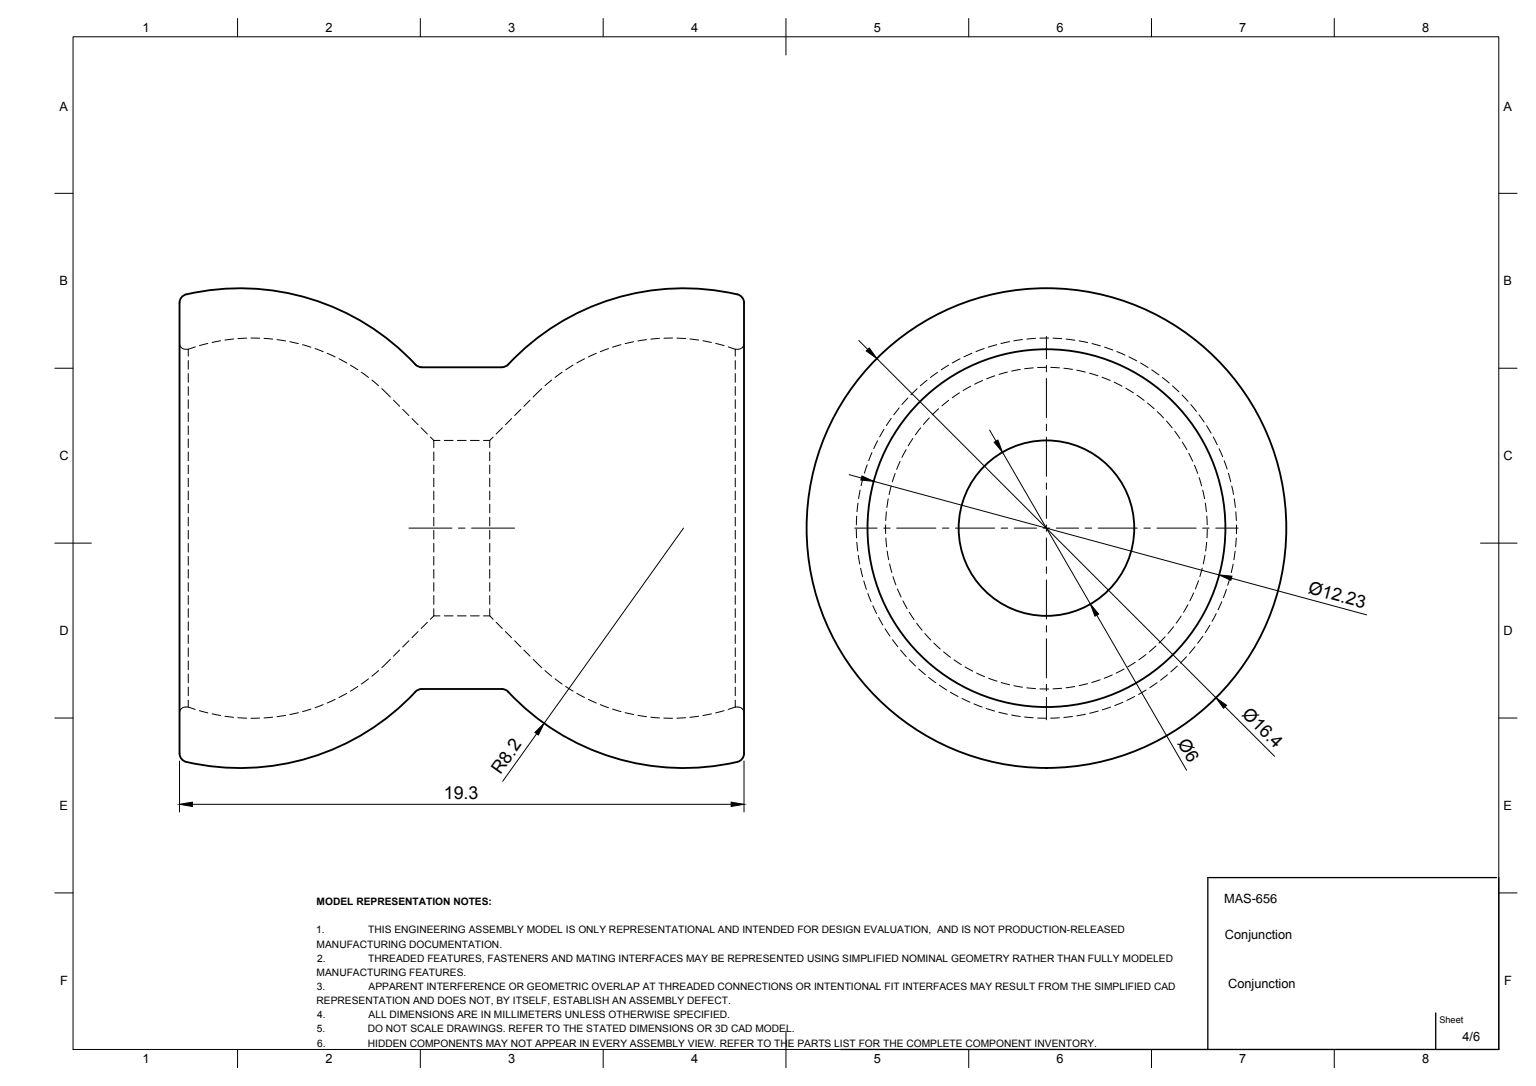
ISO-10303-21;
HEADER;
FILE_DESCRIPTION((''),'2;1');
FILE_NAME('Conjunction.step','2026-10-09T09:41:22-07:00',(''),(''),'','','');
FILE_SCHEMA (('AUTOMOTIVE_DESIGN { 1 0 10303 214 3 1 1 }'));
ENDSEC;
DATA;
#10=MECHANICAL_DESIGN_GEOMETRIC_PRESENTATION_REPRESENTATION('',(#73),#4304);
#65=SHAPE_REPRESENTATION_RELATIONSHIP('SRR','None',#4331,#69) ;
#69=ADVANCED_BREP_SHAPE_REPRESENTATION('',(#79),#4300) ;
#73=STYLED_ITEM('',(#4360),#79) ;
#79=MANIFOLD_SOLID_BREP('Body1',#2162) ;
#85=FACE_BOUND('',#630,.T.) ;
#86=FACE_BOUND('',#634,.T.) ;
#117=PLANE('',#2257) ;
#118=PLANE('',#2264) ;
#161=TOROIDAL_SURFACE('',#2228,7.69960814153059,0.300000000000023) ;
#162=TOROIDAL_SURFACE('',#2233,7.69960814153059,0.300000000000023) ;
#163=TOROIDAL_SURFACE('',#2242,5.80000000000044,0.300000000000023) ;
#164=TOROIDAL_SURFACE('',#2253,5.80000000000044,0.300000000000023) ;
#165=TOROIDAL_SURFACE('',#2259,6.31637147335048,0.200000000000015) ;
#166=TOROIDAL_SURFACE('',#2266,6.31637147335048,0.200000000000015) ;
#177=CYLINDRICAL_SURFACE('',#2221,3.00000000000023) ;
#178=CYLINDRICAL_SURFACE('',#2250,5.50000000000042) ;
#179=CYLINDRICAL_SURFACE('',#2255,6.11637147335047) ;
#180=CYLINDRICAL_SURFACE('',#2261,6.11637147335047) ;
#223=LINE('',#3294,#342) ;
#224=LINE('',#3298,#343) ;
#225=LINE('',#3301,#344) ;
#226=LINE('',#3343,#345) ;
#227=LINE('',#3351,#346) ;
#228=LINE('',#3363,#347) ;
#342=VECTOR('',#2546,3.00000000000023) ;
#343=VECTOR('',#2551,3.00000000000023) ;
#344=VECTOR('',#2554,3.00000000000023) ;
#345=VECTOR('',#2609,5.50000000000042) ;
#346=VECTOR('',#2620,6.11637147335047) ;
#347=VECTOR('',#2637,6.11637147335047) ;
#461=CONICAL_SURFACE('',#2219,3.00000000000023,0.785398163397) ;
#462=CONICAL_SURFACE('',#2223,3.00000000000023,0.785398163397) ;
#480=FACE_OUTER_BOUND('',#616,.T.) ;
#481=FACE_OUTER_BOUND('',#617,.T.) ;
#482=FACE_OUTER_BOUND('',#618,.T.) ;
#483=FACE_OUTER_BOUND('',#619,.T.) ;
#484=FACE_OUTER_BOUND('',#620,.T.) ;
#485=FACE_OUTER_BOUND('',#621,.T.) ;
#486=FACE_OUTER_BOUND('',#622,.T.) ;
#487=FACE_OUTER_BOUND('',#623,.T.) ;
#488=FACE_OUTER_BOUND('',#624,.T.) ;
#489=FACE_OUTER_BOUND('',#625,.T.) ;
#490=FACE_OUTER_BOUND('',#626,.T.) ;
#491=FACE_OUTER_BOUND('',#627,.T.) ;
#492=FACE_OUTER_BOUND('',#628,.T.) ;
#493=FACE_OUTER_BOUND('',#629,.T.) ;
#494=FACE_OUTER_BOUND('',#631,.T.) ;
#495=FACE_OUTER_BOUND('',#632,.T.) ;
#496=FACE_OUTER_BOUND('',#633,.T.) ;
#497=FACE_OUTER_BOUND('',#635,.T.) ;
#616=EDGE_LOOP('',(#1431,#1432,#1433,#1434)) ;
#617=EDGE_LOOP('',(#1435,#1436,#1437,#1438)) ;
#618=EDGE_LOOP('',(#1439,#1440,#1441,#1442)) ;
#619=EDGE_LOOP('',(#1443,#1444,#1445,#1446)) ;
#620=EDGE_LOOP('',(#1447,#1448,#1449,#1450)) ;
#621=EDGE_LOOP('',(#1451,#1452,#1453,#1454,#1455)) ;
#622=EDGE_LOOP('',(#1456,#1457,#1458,#1459,#1460)) ;
#623=EDGE_LOOP('',(#1461,#1462,#1463,#1464,#1465,#1466)) ;
#624=EDGE_LOOP('',(#1467,#1468,#1469,#1470,#1471,#1472)) ;
#625=EDGE_LOOP('',(#1473,#1474,#1475,#1476,#1477,#1478)) ;
#626=EDGE_LOOP('',(#1479,#1480,#1481,#1482,#1483,#1484)) ;
#627=EDGE_LOOP('',(#1485,#1486,#1487,#1488,#1489,#1490)) ;
#628=EDGE_LOOP('',(#1491,#1492,#1493,#1494)) ;
#629=EDGE_LOOP('',(#1495)) ;
#630=EDGE_LOOP('',(#1496)) ;
#631=EDGE_LOOP('',(#1497,#1498,#1499,#1500)) ;
#632=EDGE_LOOP('',(#1501,#1502,#1503,#1504,#1505)) ;
#633=EDGE_LOOP('',(#1506)) ;
#634=EDGE_LOOP('',(#1507)) ;
#635=EDGE_LOOP('',(#1508,#1509,#1510,#1511,#1512)) ;
#784=CIRCLE('',#2216,4.59619407771035) ;
#785=CIRCLE('',#2217,6.5000000000005) ;
#786=CIRCLE('',#2218,6.11637147335047) ;
#787=CIRCLE('',#2220,3.00000000000023) ;
#788=CIRCLE('',#2222,3.00000000000023) ;
#789=CIRCLE('',#2224,4.59619407771035) ;
#790=CIRCLE('',#2226,6.11637147335047) ;
#791=CIRCLE('',#2227,6.5000000000005) ;
#792=CIRCLE('',#2229,7.69960814153059) ;
#793=CIRCLE('',#2230,0.300000000000023) ;
#794=CIRCLE('',#2231,7.99199832412061) ;
#795=CIRCLE('',#2232,7.99199832412061) ;
#796=CIRCLE('',#2234,7.99199832412061) ;
#797=CIRCLE('',#2235,7.99199832412061) ;
#798=CIRCLE('',#2236,0.300000000000023) ;
#799=CIRCLE('',#2237,7.69960814153059) ;
#800=CIRCLE('',#2239,8.20000000000061) ;
#801=CIRCLE('',#2240,5.59529411765043) ;
#802=CIRCLE('',#2241,5.59529411765043) ;
#803=CIRCLE('',#2243,0.300000000000023) ;
#804=CIRCLE('',#2244,5.50000000000042) ;
#805=CIRCLE('',#2245,5.50000000000042) ;
#806=CIRCLE('',#2247,5.59529411765043) ;
#807=CIRCLE('',#2248,8.20000000000061) ;
#808=CIRCLE('',#2249,5.59529411765043) ;
#809=CIRCLE('',#2251,5.50000000000042) ;
#810=CIRCLE('',#2252,5.50000000000042) ;
#811=CIRCLE('',#2254,0.300000000000023) ;
#812=CIRCLE('',#2256,6.11637147335047) ;
#813=CIRCLE('',#2258,6.31637147335048) ;
#814=CIRCLE('',#2260,0.200000000000015) ;
#815=CIRCLE('',#2262,6.11637147335047) ;
#816=CIRCLE('',#2263,6.11637147335047) ;
#817=CIRCLE('',#2265,6.31637147335048) ;
#818=CIRCLE('',#2267,0.200000000000015) ;
#953=VERTEX_POINT('',#3286) ;
#954=VERTEX_POINT('',#3288) ;
#955=VERTEX_POINT('',#3292) ;
#956=VERTEX_POINT('',#3296) ;
#957=VERTEX_POINT('',#3300) ;
#958=VERTEX_POINT('',#3304) ;
#959=VERTEX_POINT('',#3308) ;
#960=VERTEX_POINT('',#3310) ;
#961=VERTEX_POINT('',#3312) ;
#962=VERTEX_POINT('',#3316) ;
#963=VERTEX_POINT('',#3317) ;
#964=VERTEX_POINT('',#3320) ;
#965=VERTEX_POINT('',#3324) ;
#966=VERTEX_POINT('',#3326) ;
#967=VERTEX_POINT('',#3330) ;
#968=VERTEX_POINT('',#3332) ;
#969=VERTEX_POINT('',#3336) ;
#970=VERTEX_POINT('',#3337) ;
#971=VERTEX_POINT('',#3342) ;
#972=VERTEX_POINT('',#3344) ;
#973=VERTEX_POINT('',#3350) ;
#974=VERTEX_POINT('',#3354) ;
#975=VERTEX_POINT('',#3359) ;
#976=VERTEX_POINT('',#3360) ;
#977=VERTEX_POINT('',#3365) ;
#1137=EDGE_CURVE('',#953,#953,#784,.T.) ;
#1138=EDGE_CURVE('',#953,#954,#785,.T.) ;
#1139=EDGE_CURVE('',#954,#954,#786,.T.) ;
#1140=EDGE_CURVE('',#955,#955,#787,.T.) ;
#1141=EDGE_CURVE('',#955,#953,#223,.T.) ;
#1142=EDGE_CURVE('',#956,#956,#788,.T.) ;
#1143=EDGE_CURVE('',#956,#955,#224,.T.) ;
#1144=EDGE_CURVE('',#956,#957,#225,.T.) ;
#1145=EDGE_CURVE('',#957,#957,#789,.F.) ;
#1146=EDGE_CURVE('',#958,#958,#790,.T.) ;
#1147=EDGE_CURVE('',#958,#957,#791,.T.) ;
#1148=EDGE_CURVE('',#959,#959,#792,.T.) ;
#1149=EDGE_CURVE('',#959,#960,#793,.T.) ;
#1150=EDGE_CURVE('',#960,#961,#794,.T.) ;
#1151=EDGE_CURVE('',#961,#960,#795,.T.) ;
#1152=EDGE_CURVE('',#962,#963,#796,.T.) ;
#1153=EDGE_CURVE('',#963,#962,#797,.T.) ;
#1154=EDGE_CURVE('',#963,#964,#798,.T.) ;
#1155=EDGE_CURVE('',#964,#964,#799,.T.) ;
#1156=EDGE_CURVE('',#961,#965,#800,.T.) ;
#1157=EDGE_CURVE('',#966,#965,#801,.F.) ;
#1158=EDGE_CURVE('',#965,#966,#802,.F.) ;
#1159=EDGE_CURVE('',#966,#967,#803,.T.) ;
#1160=EDGE_CURVE('',#968,#967,#804,.F.) ;
#1161=EDGE_CURVE('',#967,#968,#805,.F.) ;
#1162=EDGE_CURVE('',#969,#970,#806,.F.) ;
#1163=EDGE_CURVE('',#970,#962,#807,.T.) ;
#1164=EDGE_CURVE('',#970,#969,#808,.F.) ;
#1165=EDGE_CURVE('',#968,#971,#226,.T.) ;
#1166=EDGE_CURVE('',#972,#971,#809,.F.) ;
#1167=EDGE_CURVE('',#971,#972,#810,.F.) ;
#1168=EDGE_CURVE('',#972,#969,#811,.T.) ;
#1169=EDGE_CURVE('',#954,#973,#227,.T.) ;
#1170=EDGE_CURVE('',#973,#973,#812,.T.) ;
#1171=EDGE_CURVE('',#974,#974,#813,.T.) ;
#1172=EDGE_CURVE('',#973,#974,#814,.T.) ;
#1173=EDGE_CURVE('',#975,#976,#815,.T.) ;
#1174=EDGE_CURVE('',#976,#975,#816,.T.) ;
#1175=EDGE_CURVE('',#976,#958,#228,.T.) ;
#1176=EDGE_CURVE('',#977,#977,#817,.T.) ;
#1177=EDGE_CURVE('',#977,#975,#818,.T.) ;
#1431=ORIENTED_EDGE('',*,*,#1137,.F.) ;
#1432=ORIENTED_EDGE('',*,*,#1138,.T.) ;
#1433=ORIENTED_EDGE('',*,*,#1139,.T.) ;
#1434=ORIENTED_EDGE('',*,*,#1138,.F.) ;
#1435=ORIENTED_EDGE('',*,*,#1140,.F.) ;
#1436=ORIENTED_EDGE('',*,*,#1141,.T.) ;
#1437=ORIENTED_EDGE('',*,*,#1137,.T.) ;
#1438=ORIENTED_EDGE('',*,*,#1141,.F.) ;
#1439=ORIENTED_EDGE('',*,*,#1142,.F.) ;
#1440=ORIENTED_EDGE('',*,*,#1143,.T.) ;
#1441=ORIENTED_EDGE('',*,*,#1140,.T.) ;
#1442=ORIENTED_EDGE('',*,*,#1143,.F.) ;
#1443=ORIENTED_EDGE('',*,*,#1142,.T.) ;
#1444=ORIENTED_EDGE('',*,*,#1144,.T.) ;
#1445=ORIENTED_EDGE('',*,*,#1145,.F.) ;
#1446=ORIENTED_EDGE('',*,*,#1144,.F.) ;
#1447=ORIENTED_EDGE('',*,*,#1146,.F.) ;
#1448=ORIENTED_EDGE('',*,*,#1147,.T.) ;
#1449=ORIENTED_EDGE('',*,*,#1145,.T.) ;
#1450=ORIENTED_EDGE('',*,*,#1147,.F.) ;
#1451=ORIENTED_EDGE('',*,*,#1148,.F.) ;
#1452=ORIENTED_EDGE('',*,*,#1149,.T.) ;
#1453=ORIENTED_EDGE('',*,*,#1150,.T.) ;
#1454=ORIENTED_EDGE('',*,*,#1151,.T.) ;
#1455=ORIENTED_EDGE('',*,*,#1149,.F.) ;
#1456=ORIENTED_EDGE('',*,*,#1152,.F.) ;
#1457=ORIENTED_EDGE('',*,*,#1153,.F.) ;
#1458=ORIENTED_EDGE('',*,*,#1154,.T.) ;
#1459=ORIENTED_EDGE('',*,*,#1155,.T.) ;
#1460=ORIENTED_EDGE('',*,*,#1154,.F.) ;
#1461=ORIENTED_EDGE('',*,*,#1151,.F.) ;
#1462=ORIENTED_EDGE('',*,*,#1156,.T.) ;
#1463=ORIENTED_EDGE('',*,*,#1157,.F.) ;
#1464=ORIENTED_EDGE('',*,*,#1158,.F.) ;
#1465=ORIENTED_EDGE('',*,*,#1156,.F.) ;
#1466=ORIENTED_EDGE('',*,*,#1150,.F.) ;
#1467=ORIENTED_EDGE('',*,*,#1157,.T.) ;
#1468=ORIENTED_EDGE('',*,*,#1158,.T.) ;
#1469=ORIENTED_EDGE('',*,*,#1159,.T.) ;
#1470=ORIENTED_EDGE('',*,*,#1160,.F.) ;
#1471=ORIENTED_EDGE('',*,*,#1161,.F.) ;
#1472=ORIENTED_EDGE('',*,*,#1159,.F.) ;
#1473=ORIENTED_EDGE('',*,*,#1162,.T.) ;
#1474=ORIENTED_EDGE('',*,*,#1163,.T.) ;
#1475=ORIENTED_EDGE('',*,*,#1152,.T.) ;
#1476=ORIENTED_EDGE('',*,*,#1153,.T.) ;
#1477=ORIENTED_EDGE('',*,*,#1163,.F.) ;
#1478=ORIENTED_EDGE('',*,*,#1164,.T.) ;
#1479=ORIENTED_EDGE('',*,*,#1160,.T.) ;
#1480=ORIENTED_EDGE('',*,*,#1161,.T.) ;
#1481=ORIENTED_EDGE('',*,*,#1165,.T.) ;
#1482=ORIENTED_EDGE('',*,*,#1166,.F.) ;
#1483=ORIENTED_EDGE('',*,*,#1167,.F.) ;
#1484=ORIENTED_EDGE('',*,*,#1165,.F.) ;
#1485=ORIENTED_EDGE('',*,*,#1166,.T.) ;
#1486=ORIENTED_EDGE('',*,*,#1167,.T.) ;
#1487=ORIENTED_EDGE('',*,*,#1168,.T.) ;
#1488=ORIENTED_EDGE('',*,*,#1164,.F.) ;
#1489=ORIENTED_EDGE('',*,*,#1162,.F.) ;
#1490=ORIENTED_EDGE('',*,*,#1168,.F.) ;
#1491=ORIENTED_EDGE('',*,*,#1139,.F.) ;
#1492=ORIENTED_EDGE('',*,*,#1169,.T.) ;
#1493=ORIENTED_EDGE('',*,*,#1170,.T.) ;
#1494=ORIENTED_EDGE('',*,*,#1169,.F.) ;
#1495=ORIENTED_EDGE('',*,*,#1148,.T.) ;
#1496=ORIENTED_EDGE('',*,*,#1171,.F.) ;
#1497=ORIENTED_EDGE('',*,*,#1170,.F.) ;
#1498=ORIENTED_EDGE('',*,*,#1172,.T.) ;
#1499=ORIENTED_EDGE('',*,*,#1171,.T.) ;
#1500=ORIENTED_EDGE('',*,*,#1172,.F.) ;
#1501=ORIENTED_EDGE('',*,*,#1173,.F.) ;
#1502=ORIENTED_EDGE('',*,*,#1174,.F.) ;
#1503=ORIENTED_EDGE('',*,*,#1175,.T.) ;
#1504=ORIENTED_EDGE('',*,*,#1146,.T.) ;
#1505=ORIENTED_EDGE('',*,*,#1175,.F.) ;
#1506=ORIENTED_EDGE('',*,*,#1155,.F.) ;
#1507=ORIENTED_EDGE('',*,*,#1176,.T.) ;
#1508=ORIENTED_EDGE('',*,*,#1176,.F.) ;
#1509=ORIENTED_EDGE('',*,*,#1177,.T.) ;
#1510=ORIENTED_EDGE('',*,*,#1173,.T.) ;
#1511=ORIENTED_EDGE('',*,*,#1174,.T.) ;
#1512=ORIENTED_EDGE('',*,*,#1177,.F.) ;
#2019=SPHERICAL_SURFACE('',#2215,6.5000000000005) ;
#2020=SPHERICAL_SURFACE('',#2225,6.5000000000005) ;
#2021=SPHERICAL_SURFACE('',#2238,8.20000000000063) ;
#2022=SPHERICAL_SURFACE('',#2246,8.20000000000063) ;
#2026=ADVANCED_FACE('',(#480),#2019,.F.) ;
#2027=ADVANCED_FACE('',(#481),#461,.F.) ;
#2028=ADVANCED_FACE('',(#482),#177,.F.) ;
#2029=ADVANCED_FACE('',(#483),#462,.F.) ;
#2030=ADVANCED_FACE('',(#484),#2020,.F.) ;
#2031=ADVANCED_FACE('',(#485),#161,.T.) ;
#2032=ADVANCED_FACE('',(#486),#162,.T.) ;
#2033=ADVANCED_FACE('',(#487),#2021,.T.) ;
#2034=ADVANCED_FACE('',(#488),#163,.F.) ;
#2035=ADVANCED_FACE('',(#489),#2022,.T.) ;
#2036=ADVANCED_FACE('',(#490),#178,.T.) ;
#2037=ADVANCED_FACE('',(#491),#164,.F.) ;
#2038=ADVANCED_FACE('',(#492),#179,.F.) ;
#2039=ADVANCED_FACE('',(#493,#85),#117,.T.) ;
#2040=ADVANCED_FACE('',(#494),#165,.T.) ;
#2041=ADVANCED_FACE('',(#495),#180,.F.) ;
#2042=ADVANCED_FACE('',(#496,#86),#118,.F.) ;
#2043=ADVANCED_FACE('',(#497),#166,.T.) ;
#2162=CLOSED_SHELL('',(#2026,#2027,#2028,#2029,#2030,#2031,#2032,#2033,
#2034,#2035,#2036,#2037,#2038,#2039,#2040,#2041,#2042,#2043)) ;
#2214=AXIS2_PLACEMENT_3D('',#3284,#2532,#2533) ;
#2215=AXIS2_PLACEMENT_3D('',#3285,#2534,#2535) ;
#2216=AXIS2_PLACEMENT_3D('',#3287,#2536,#2537) ;
#2217=AXIS2_PLACEMENT_3D('',#3289,#2538,#2539) ;
#2218=AXIS2_PLACEMENT_3D('',#3290,#2540,#2541) ;
#2219=AXIS2_PLACEMENT_3D('',#3291,#2542,#2543) ;
#2220=AXIS2_PLACEMENT_3D('',#3293,#2544,#2545) ;
#2221=AXIS2_PLACEMENT_3D('',#3295,#2547,#2548) ;
#2222=AXIS2_PLACEMENT_3D('',#3297,#2549,#2550) ;
#2223=AXIS2_PLACEMENT_3D('',#3299,#2552,#2553) ;
#2224=AXIS2_PLACEMENT_3D('',#3302,#2555,#2556) ;
#2225=AXIS2_PLACEMENT_3D('',#3303,#2557,#2558) ;
#2226=AXIS2_PLACEMENT_3D('',#3305,#2559,#2560) ;
#2227=AXIS2_PLACEMENT_3D('',#3306,#2561,#2562) ;
#2228=AXIS2_PLACEMENT_3D('',#3307,#2563,#2564) ;
#2229=AXIS2_PLACEMENT_3D('',#3309,#2565,#2566) ;
#2230=AXIS2_PLACEMENT_3D('',#3311,#2567,#2568) ;
#2231=AXIS2_PLACEMENT_3D('',#3313,#2569,#2570) ;
#2232=AXIS2_PLACEMENT_3D('',#3314,#2571,#2572) ;
#2233=AXIS2_PLACEMENT_3D('',#3315,#2573,#2574) ;
#2234=AXIS2_PLACEMENT_3D('',#3318,#2575,#2576) ;
#2235=AXIS2_PLACEMENT_3D('',#3319,#2577,#2578) ;
#2236=AXIS2_PLACEMENT_3D('',#3321,#2579,#2580) ;
#2237=AXIS2_PLACEMENT_3D('',#3322,#2581,#2582) ;
#2238=AXIS2_PLACEMENT_3D('',#3323,#2583,#2584) ;
#2239=AXIS2_PLACEMENT_3D('',#3325,#2585,#2586) ;
#2240=AXIS2_PLACEMENT_3D('',#3327,#2587,#2588) ;
#2241=AXIS2_PLACEMENT_3D('',#3328,#2589,#2590) ;
#2242=AXIS2_PLACEMENT_3D('',#3329,#2591,#2592) ;
#2243=AXIS2_PLACEMENT_3D('',#3331,#2593,#2594) ;
#2244=AXIS2_PLACEMENT_3D('',#3333,#2595,#2596) ;
#2245=AXIS2_PLACEMENT_3D('',#3334,#2597,#2598) ;
#2246=AXIS2_PLACEMENT_3D('',#3335,#2599,#2600) ;
#2247=AXIS2_PLACEMENT_3D('',#3338,#2601,#2602) ;
#2248=AXIS2_PLACEMENT_3D('',#3339,#2603,#2604) ;
#2249=AXIS2_PLACEMENT_3D('',#3340,#2605,#2606) ;
#2250=AXIS2_PLACEMENT_3D('',#3341,#2607,#2608) ;
#2251=AXIS2_PLACEMENT_3D('',#3345,#2610,#2611) ;
#2252=AXIS2_PLACEMENT_3D('',#3346,#2612,#2613) ;
#2253=AXIS2_PLACEMENT_3D('',#3347,#2614,#2615) ;
#2254=AXIS2_PLACEMENT_3D('',#3348,#2616,#2617) ;
#2255=AXIS2_PLACEMENT_3D('',#3349,#2618,#2619) ;
#2256=AXIS2_PLACEMENT_3D('',#3352,#2621,#2622) ;
#2257=AXIS2_PLACEMENT_3D('',#3353,#2623,#2624) ;
#2258=AXIS2_PLACEMENT_3D('',#3355,#2625,#2626) ;
#2259=AXIS2_PLACEMENT_3D('',#3356,#2627,#2628) ;
#2260=AXIS2_PLACEMENT_3D('',#3357,#2629,#2630) ;
#2261=AXIS2_PLACEMENT_3D('',#3358,#2631,#2632) ;
#2262=AXIS2_PLACEMENT_3D('',#3361,#2633,#2634) ;
#2263=AXIS2_PLACEMENT_3D('',#3362,#2635,#2636) ;
#2264=AXIS2_PLACEMENT_3D('',#3364,#2638,#2639) ;
#2265=AXIS2_PLACEMENT_3D('',#3366,#2640,#2641) ;
#2266=AXIS2_PLACEMENT_3D('',#3367,#2642,#2643) ;
#2267=AXIS2_PLACEMENT_3D('',#3368,#2644,#2645) ;
#2532=DIRECTION('axis',(0.,0.,1.)) ;
#2533=DIRECTION('refdir',(1.,0.,0.)) ;
#2534=DIRECTION('center_axis',(0.855521240266964,-0.510121382366095,0.0886542875724551)) ;
#2535=DIRECTION('ref_axis',(-0.465119843688757,-0.832406937999121,-0.301267689236458)) ;
#2536=DIRECTION('center_axis',(0.855521240266964,-0.510121382366096,0.0886542875724545)) ;
#2537=DIRECTION('ref_axis',(-0.517240562193751,-0.834304337432909,0.190783839363105)) ;
#2538=DIRECTION('center_axis',(0.227479534154222,0.216506038769898,-0.949409393632244)) ;
#2539=DIRECTION('ref_axis',(0.465119843688755,0.832406937999122,0.301267689236458)) ;
#2540=DIRECTION('center_axis',(0.855521240266964,-0.510121382366096,0.0886542875724545)) ;
#2541=DIRECTION('ref_axis',(-0.517240562193751,-0.834304337432909,0.190783839363105)) ;
#2542=DIRECTION('center_axis',(0.855521240266964,-0.510121382366096,0.0886542875724545)) ;
#2543=DIRECTION('ref_axis',(-0.465119843688758,-0.83240693799912,-0.301267689236458)) ;
#2544=DIRECTION('center_axis',(0.855521240266964,-0.510121382366096,0.0886542875724545)) ;
#2545=DIRECTION('ref_axis',(-0.517240562193751,-0.834304337432909,0.190783839363105)) ;
#2546=DIRECTION('',(0.933834265978767,0.22789030186616,0.275716473935178)) ;
#2547=DIRECTION('center_axis',(0.855521240266964,-0.510121382366096,0.0886542875724545)) ;
#2548=DIRECTION('ref_axis',(-0.465119843688758,-0.83240693799912,-0.301267689236458)) ;
#2549=DIRECTION('center_axis',(0.855521240266964,-0.510121382366096,0.0886542875724545)) ;
#2550=DIRECTION('ref_axis',(-0.517240562193751,-0.834304337432909,0.190783839363105)) ;
#2551=DIRECTION('',(0.855521240266964,-0.510121382366096,0.0886542875724545)) ;
#2552=DIRECTION('center_axis',(-0.855521240266964,0.510121382366096,-0.0886542875724545)) ;
#2553=DIRECTION('ref_axis',(-0.465119843688758,-0.83240693799912,-0.301267689236458)) ;
#2554=DIRECTION('',(-0.276055474905567,0.949310879265128,0.150340378087632)) ;
#2555=DIRECTION('center_axis',(-0.855521240266964,0.510121382366096,-0.0886542875724545)) ;
#2556=DIRECTION('ref_axis',(0.517240562193751,0.834304337432909,-0.190783839363105)) ;
#2557=DIRECTION('center_axis',(0.855521240266964,-0.510121382366095,0.0886542875724551)) ;
#2558=DIRECTION('ref_axis',(-0.465119843688757,-0.832406937999121,-0.301267689236458)) ;
#2559=DIRECTION('center_axis',(0.855521240266964,-0.510121382366096,0.0886542875724545)) ;
#2560=DIRECTION('ref_axis',(-0.517240562193751,-0.834304337432909,0.190783839363105)) ;
#2561=DIRECTION('center_axis',(0.227479534154222,0.216506038769898,-0.949409393632244)) ;
#2562=DIRECTION('ref_axis',(0.465119843688755,0.832406937999122,0.301267689236458)) ;
#2563=DIRECTION('center_axis',(0.855521240266964,-0.510121382366096,0.0886542875724545)) ;
#2564=DIRECTION('ref_axis',(0.517704809501169,0.845453579256405,-0.131110547027658)) ;
#2565=DIRECTION('center_axis',(0.855521240266964,-0.510121382366096,0.0886542875724545)) ;
#2566=DIRECTION('ref_axis',(-0.517240562193751,-0.834304337432909,0.190783839363105)) ;
#2567=DIRECTION('center_axis',(0.00807079125203423,-0.158064608864342,-0.987395787793896)) ;
#2568=DIRECTION('ref_axis',(-0.517704809501169,-0.845453579256405,0.131110547027658)) ;
#2569=DIRECTION('center_axis',(0.855521240266964,-0.510121382366096,0.0886542875724545)) ;
#2570=DIRECTION('ref_axis',(-0.517240562193751,-0.834304337432909,0.190783839363105)) ;
#2571=DIRECTION('center_axis',(0.855521240266964,-0.510121382366096,0.0886542875724545)) ;
#2572=DIRECTION('ref_axis',(-0.517240562193751,-0.834304337432909,0.190783839363105)) ;
#2573=DIRECTION('center_axis',(0.855521240266964,-0.510121382366096,0.0886542875724545)) ;
#2574=DIRECTION('ref_axis',(0.486257491979136,0.850411106325231,0.20088454826805)) ;
#2575=DIRECTION('center_axis',(0.855521240266964,-0.510121382366096,0.0886542875724545)) ;
#2576=DIRECTION('ref_axis',(-0.517240562193751,-0.834304337432909,0.190783839363105)) ;
#2577=DIRECTION('center_axis',(0.855521240266964,-0.510121382366096,0.0886542875724545)) ;
#2578=DIRECTION('ref_axis',(-0.517240562193751,-0.834304337432909,0.190783839363105)) ;
#2579=DIRECTION('center_axis',(0.177868094233453,0.128752186356572,-0.975595108414429)) ;
#2580=DIRECTION('ref_axis',(-0.486257491979132,-0.850411106325233,-0.20088454826805)) ;
#2581=DIRECTION('center_axis',(0.855521240266964,-0.510121382366096,0.0886542875724545)) ;
#2582=DIRECTION('ref_axis',(-0.517240562193751,-0.834304337432909,0.190783839363105)) ;
#2583=DIRECTION('center_axis',(0.855521240266964,-0.510121382366096,0.0886542875724545)) ;
#2584=DIRECTION('ref_axis',(-0.465119843688757,-0.83240693799912,-0.301267689236459)) ;
#2585=DIRECTION('center_axis',(-0.227479534154222,-0.2165060387699,0.949409393632244)) ;
#2586=DIRECTION('ref_axis',(0.465119843688754,0.832406937999121,0.301267689236459)) ;
#2587=DIRECTION('center_axis',(0.855521240266964,-0.510121382366096,0.0886542875724545)) ;
#2588=DIRECTION('ref_axis',(-0.517240562193751,-0.834304337432909,0.190783839363105)) ;
#2589=DIRECTION('center_axis',(0.855521240266964,-0.510121382366096,0.0886542875724545)) ;
#2590=DIRECTION('ref_axis',(-0.517240562193751,-0.834304337432909,0.190783839363105)) ;
#2591=DIRECTION('center_axis',(0.855521240266964,-0.510121382366096,0.0886542875724545)) ;
#2592=DIRECTION('ref_axis',(0.509998973339442,0.800690415698108,-0.314318159516605)) ;
#2593=DIRECTION('center_axis',(0.0893557756655694,0.314119457312167,0.945169038793122)) ;
#2594=DIRECTION('ref_axis',(-0.509998973339435,-0.800690415698112,0.314318159516606)) ;
#2595=DIRECTION('center_axis',(0.855521240266964,-0.510121382366096,0.0886542875724545)) ;
#2596=DIRECTION('ref_axis',(-0.517240562193751,-0.834304337432909,0.190783839363105)) ;
#2597=DIRECTION('center_axis',(0.855521240266964,-0.510121382366096,0.0886542875724545)) ;
#2598=DIRECTION('ref_axis',(-0.517240562193751,-0.834304337432909,0.190783839363105)) ;
#2599=DIRECTION('center_axis',(0.855521240266964,-0.510121382366096,0.0886542875724545)) ;
#2600=DIRECTION('ref_axis',(-0.465119843688757,-0.83240693799912,-0.301267689236459)) ;
#2601=DIRECTION('center_axis',(0.855521240266964,-0.510121382366096,0.0886542875724545)) ;
#2602=DIRECTION('ref_axis',(-0.517240562193751,-0.834304337432909,0.190783839363105)) ;
#2603=DIRECTION('center_axis',(-0.227479534154222,-0.2165060387699,0.949409393632244)) ;
#2604=DIRECTION('ref_axis',(0.465119843688754,0.832406937999121,0.301267689236459)) ;
#2605=DIRECTION('center_axis',(0.855521240266964,-0.510121382366096,0.0886542875724545)) ;
#2606=DIRECTION('ref_axis',(-0.517240562193751,-0.834304337432909,0.190783839363105)) ;
#2607=DIRECTION('center_axis',(0.855521240266964,-0.510121382366096,0.0886542875724545)) ;
#2608=DIRECTION('ref_axis',(-0.465119843688758,-0.83240693799912,-0.301267689236458)) ;
#2609=DIRECTION('',(-0.855521240266964,0.510121382366096,-0.0886542875724545)) ;
#2610=DIRECTION('center_axis',(0.855521240266964,-0.510121382366096,0.0886542875724545)) ;
#2611=DIRECTION('ref_axis',(-0.517240562193751,-0.834304337432909,0.190783839363105)) ;
#2612=DIRECTION('center_axis',(0.855521240266964,-0.510121382366096,0.0886542875724545)) ;
#2613=DIRECTION('ref_axis',(-0.517240562193751,-0.834304337432909,0.190783839363105)) ;
#2614=DIRECTION('center_axis',(0.855521240266964,-0.510121382366096,0.0886542875724545)) ;
#2615=DIRECTION('ref_axis',(0.509998973339442,0.800690415698108,-0.314318159516605)) ;
#2616=DIRECTION('center_axis',(0.0893557756655694,0.314119457312167,0.945169038793122)) ;
#2617=DIRECTION('ref_axis',(-0.509998973339435,-0.800690415698112,0.314318159516606)) ;
#2618=DIRECTION('center_axis',(0.855521240266964,-0.510121382366096,0.0886542875724545)) ;
#2619=DIRECTION('ref_axis',(-0.465119843688758,-0.83240693799912,-0.301267689236458)) ;
#2620=DIRECTION('',(0.855521240266964,-0.510121382366096,0.0886542875724545)) ;
#2621=DIRECTION('center_axis',(0.855521240266964,-0.510121382366096,0.0886542875724545)) ;
#2622=DIRECTION('ref_axis',(-0.517240562193751,-0.834304337432909,0.190783839363105)) ;
#2623=DIRECTION('center_axis',(0.855521240266964,-0.510121382366096,0.0886542875724545)) ;
#2624=DIRECTION('ref_axis',(0.0233582592152953,0.20907522041968,0.977620552122803)) ;
#2625=DIRECTION('center_axis',(0.855521240266964,-0.510121382366096,0.0886542875724545)) ;
#2626=DIRECTION('ref_axis',(-0.517240562193751,-0.834304337432909,0.190783839363105)) ;
#2627=DIRECTION('center_axis',(0.855521240266964,-0.510121382366096,0.0886542875724545)) ;
#2628=DIRECTION('ref_axis',(-0.465119843688758,-0.83240693799912,-0.301267689236458)) ;
#2629=DIRECTION('center_axis',(-0.227479534154222,-0.216506038769899,0.949409393632244)) ;
#2630=DIRECTION('ref_axis',(0.465119843688755,0.832406937999121,0.301267689236459)) ;
#2631=DIRECTION('center_axis',(0.855521240266964,-0.510121382366096,0.0886542875724545)) ;
#2632=DIRECTION('ref_axis',(-0.465119843688758,-0.83240693799912,-0.301267689236458)) ;
#2633=DIRECTION('center_axis',(0.855521240266964,-0.510121382366096,0.0886542875724545)) ;
#2634=DIRECTION('ref_axis',(-0.517240562193751,-0.834304337432909,0.190783839363105)) ;
#2635=DIRECTION('center_axis',(0.855521240266964,-0.510121382366096,0.0886542875724545)) ;
#2636=DIRECTION('ref_axis',(-0.517240562193751,-0.834304337432909,0.190783839363105)) ;
#2637=DIRECTION('',(0.855521240266964,-0.510121382366096,0.0886542875724545)) ;
#2638=DIRECTION('center_axis',(0.855521240266964,-0.510121382366096,0.0886542875724545)) ;
#2639=DIRECTION('ref_axis',(0.0233582592152953,0.20907522041968,0.977620552122803)) ;
#2640=DIRECTION('center_axis',(0.855521240266964,-0.510121382366096,0.0886542875724545)) ;
#2641=DIRECTION('ref_axis',(-0.517240562193751,-0.834304337432909,0.190783839363105)) ;
#2642=DIRECTION('center_axis',(0.855521240266963,-0.510121382366096,0.0886542875724557)) ;
#2643=DIRECTION('ref_axis',(0.484971795675454,0.849467667676745,0.207863029351437)) ;
#2644=DIRECTION('center_axis',(0.181344326769277,0.134836407638048,-0.974132115436024)) ;
#2645=DIRECTION('ref_axis',(-0.484971795675455,-0.849467667676745,-0.207863029351437)) ;
#3284=CARTESIAN_POINT('',(0.,0.,0.)) ;
#3285=CARTESIAN_POINT('Origin',(-434.543858273742,156.789736278414,-59.8178313623822)) ;
#3286=CARTESIAN_POINT('',(-436.338218860625,162.960256993635,-58.8406189048122)) ;
#3287=CARTESIAN_POINT('Origin',(-438.475999931612,159.134353154959,-60.2253036738863)) ;
#3288=CARTESIAN_POINT('',(-429.816865801527,160.758779287006,-57.7801268294347)) ;
#3289=CARTESIAN_POINT('Origin',(-434.543858273742,156.789736278414,-59.8178313623822)) ;
#3290=CARTESIAN_POINT('Origin',(-432.661711545155,155.667469237209,-59.6227919297228)) ;
#3291=CARTESIAN_POINT('Origin',(-439.841577868686,159.948605884407,-60.3668131226735)) ;
#3292=CARTESIAN_POINT('',(-438.44621833762,162.445826698405,-59.4630100549641)) ;
#3293=CARTESIAN_POINT('Origin',(-439.841577868686,159.948605884407,-60.3668131226735)) ;
#3294=CARTESIAN_POINT('',(-438.44621833762,162.445826698405,-59.4630100549641)) ;
#3295=CARTESIAN_POINT('Origin',(-440.660835141651,160.437104162332,-60.4517095185253)) ;
#3296=CARTESIAN_POINT('',(-440.08473288355,163.422823254255,-59.6328028466676)) ;
#3297=CARTESIAN_POINT('Origin',(-441.480092414616,160.925602440257,-60.536605914377)) ;
#3298=CARTESIAN_POINT('',(-439.265475610585,162.93432497633,-59.5479064508159)) ;
#3299=CARTESIAN_POINT('Origin',(-441.480092414616,160.925602440257,-60.536605914377)) ;
#3300=CARTESIAN_POINT('',(-440.7078892807,165.565759008383,-59.2934305940894)) ;
#3301=CARTESIAN_POINT('',(-440.08473288355,163.422823254255,-59.6328028466676)) ;
#3302=CARTESIAN_POINT('Origin',(-442.84567035169,161.739855169706,-60.6781153631642)) ;
#3303=CARTESIAN_POINT('Origin',(-446.77781200956,164.08447204625,-61.0855876746684)) ;
#3304=CARTESIAN_POINT('',(-445.815112994521,170.298049137252,-59.4379620070397)) ;
#3305=CARTESIAN_POINT('Origin',(-448.659958738148,165.206739087456,-61.2806271073278)) ;
#3306=CARTESIAN_POINT('Origin',(-446.77781200956,164.08447204625,-61.0855876746684)) ;
#3307=CARTESIAN_POINT('Origin',(-432.661711545155,155.667469237209,-59.6227919297228)) ;
#3308=CARTESIAN_POINT('',(-436.391179339219,149.00477156037,-58.5866958081163)) ;
#3309=CARTESIAN_POINT('Origin',(-432.405055173074,155.514432822499,-59.596195643451)) ;
#3310=CARTESIAN_POINT('',(-436.741766535065,148.876355333483,-58.5690042756859)) ;
#3311=CARTESIAN_POINT('Origin',(-436.6478357113,149.15780797508,-58.6132920943881)) ;
#3312=CARTESIAN_POINT('',(-428.887033553867,162.285813775497,-57.209108680316)) ;
#3313=CARTESIAN_POINT('Origin',(-432.604270565142,155.633218922022,-59.6168395478055)) ;
#3314=CARTESIAN_POINT('Origin',(-432.604270565142,155.633218922022,-59.6168395478055)) ;
#3315=CARTESIAN_POINT('Origin',(-448.659958738148,165.206739087456,-61.2806271073278)) ;
#3316=CARTESIAN_POINT('',(-445.000162706884,171.893584256118,-58.8788486217556)) ;
#3317=CARTESIAN_POINT('',(-452.603568779148,158.444505266078,-62.892048462345)) ;
#3318=CARTESIAN_POINT('Origin',(-448.71739971816,165.240989402643,-61.2865794892451)) ;
#3319=CARTESIAN_POINT('Origin',(-448.71739971816,165.240989402643,-61.2865794892451)) ;
#3320=CARTESIAN_POINT('',(-452.660607254351,158.811943224256,-62.8539556969519)) ;
#3321=CARTESIAN_POINT('Origin',(-452.403950882271,158.658906809546,-62.8273594106802)) ;
#3322=CARTESIAN_POINT('Origin',(-448.916615110228,165.359775502165,-61.3072233935995)) ;
#3323=CARTESIAN_POINT('Origin',(-434.174324018733,156.569394203754,-59.7795379868709)) ;
#3324=CARTESIAN_POINT('',(-436.700167681604,164.284821180549,-58.625284827235)) ;
#3325=CARTESIAN_POINT('Origin',(-434.174324018733,156.569394203754,-59.7795379868709)) ;
#3326=CARTESIAN_POINT('',(-442.156244262532,155.147161163856,-58.5522636076438)) ;
#3327=CARTESIAN_POINT('Origin',(-439.302650006998,159.627259536871,-60.3109661566578)) ;
#3328=CARTESIAN_POINT('Origin',(-439.302650006998,159.627259536871,-60.3109661566578)) ;
#3329=CARTESIAN_POINT('Origin',(-439.490271689493,159.739132658813,-60.3304086506742)) ;
#3330=CARTESIAN_POINT('',(-442.29526604286,155.335335372473,-58.6016587733327)) ;
#3331=CARTESIAN_POINT('Origin',(-442.448265734862,155.095128247764,-58.5073633254777)) ;
#3332=CARTESIAN_POINT('',(-436.932112549205,164.317370817808,-58.6734363598735)) ;
#3333=CARTESIAN_POINT('Origin',(-439.490271689493,159.739132658813,-60.3304086506742)) ;
#3334=CARTESIAN_POINT('Origin',(-439.490271689493,159.739132658813,-60.3304086506742)) ;
#3335=CARTESIAN_POINT('Origin',(-447.147346264569,164.304814120911,-61.1238810501796)) ;
#3336=CARTESIAN_POINT('',(-444.872614531839,156.766850414779,-58.8337503313788)) ;
#3337=CARTESIAN_POINT('',(-439.416537950911,165.904510431472,-58.9067715509699)) ;
#3338=CARTESIAN_POINT('Origin',(-442.019020276305,161.246948787794,-60.5924528803928)) ;
#3339=CARTESIAN_POINT('Origin',(-447.147346264569,164.304814120911,-61.1238810501796)) ;
#3340=CARTESIAN_POINT('Origin',(-442.019020276305,161.246948787794,-60.5924528803928)) ;
#3341=CARTESIAN_POINT('Origin',(-440.660835141651,160.437104162332,-60.4517095185253)) ;
#3342=CARTESIAN_POINT('',(-439.273239453521,165.713313824847,-58.9160380955758)) ;
#3343=CARTESIAN_POINT('',(-438.102676001363,165.015342321328,-58.7947372277247)) ;
#3344=CARTESIAN_POINT('',(-444.636392947176,156.731278379512,-58.8442605090349)) ;
#3345=CARTESIAN_POINT('Origin',(-441.831398593809,161.135075665852,-60.5730103863764)) ;
#3346=CARTESIAN_POINT('Origin',(-441.831398593809,161.135075665852,-60.5730103863764)) ;
#3347=CARTESIAN_POINT('Origin',(-441.831398593809,161.135075665852,-60.5730103863764)) ;
#3348=CARTESIAN_POINT('Origin',(-444.789392639178,156.491071254803,-58.7499650611799)) ;
#3349=CARTESIAN_POINT('Origin',(-440.660835141651,160.437104162332,-60.4517095185253)) ;
#3350=CARTESIAN_POINT('',(-429.731313677501,160.707767148769,-57.7712614006774)) ;
#3351=CARTESIAN_POINT('',(-437.815989398024,165.528414212129,-58.6090444182372)) ;
#3352=CARTESIAN_POINT('Origin',(-432.576159421128,155.616457098972,-59.6139265009655)) ;
#3353=CARTESIAN_POINT('Origin',(-436.509323339471,148.894285480052,-58.0823390440383)) ;
#3354=CARTESIAN_POINT('',(-429.46718544632,160.77222427359,-57.6932770653741)) ;
#3355=CARTESIAN_POINT('Origin',(-432.405055173074,155.514432822499,-59.596195643451)) ;
#3356=CARTESIAN_POINT('Origin',(-432.576159421128,155.616457098972,-59.6139265009655)) ;
#3357=CARTESIAN_POINT('Origin',(-429.638289708763,160.874248536369,-57.7110078628301)) ;
#3358=CARTESIAN_POINT('Origin',(-440.660835141651,160.437104162332,-60.4517095185253)) ;
#3359=CARTESIAN_POINT('',(-451.711778518624,160.062091415581,-62.5608600391744)) ;
#3360=CARTESIAN_POINT('',(-445.900665118548,170.349061275489,-59.446827435797)) ;
#3361=CARTESIAN_POINT('Origin',(-448.745510862175,165.257751225692,-61.289492536085)) ;
#3362=CARTESIAN_POINT('Origin',(-448.745510862175,165.257751225692,-61.289492536085)) ;
#3363=CARTESIAN_POINT('',(-437.815989398024,165.528414212129,-58.6090444182372)) ;
#3364=CARTESIAN_POINT('Origin',(-453.020883276625,158.739628159719,-59.7933667941868)) ;
#3365=CARTESIAN_POINT('',(-451.979877125812,159.994222158519,-62.6201635025592)) ;
#3366=CARTESIAN_POINT('Origin',(-448.916615110228,165.359775502165,-61.3072233935995)) ;
#3367=CARTESIAN_POINT('Origin',(-448.745510862175,165.257751225692,-61.289492536085)) ;
#3368=CARTESIAN_POINT('Origin',(-451.808772877759,159.892197882045,-62.6024326450446)) ;
#4294=UNCERTAINTY_MEASURE_WITH_UNIT(LENGTH_MEASURE(0.01),#4305,
'DISTANCE_ACCURACY_VALUE',
'Maximum model space distance between geometric entities at asserted c
onnectivities') ;
#4298=UNCERTAINTY_MEASURE_WITH_UNIT(LENGTH_MEASURE(0.01),#4305,
'DISTANCE_ACCURACY_VALUE',
'Maximum model space distance between geometric entities at asserted c
onnectivities') ;
#4300=(
GEOMETRIC_REPRESENTATION_CONTEXT(3)
GLOBAL_UNCERTAINTY_ASSIGNED_CONTEXT((#4294))
GLOBAL_UNIT_ASSIGNED_CONTEXT((#4305,#4307,#4308))
REPRESENTATION_CONTEXT('','3D')
) ;
#4304=(
GEOMETRIC_REPRESENTATION_CONTEXT(3)
GLOBAL_UNCERTAINTY_ASSIGNED_CONTEXT((#4298))
GLOBAL_UNIT_ASSIGNED_CONTEXT((#4305,#4307,#4308))
REPRESENTATION_CONTEXT('','3D')
) ;
#4305=(
LENGTH_UNIT()
NAMED_UNIT(*)
SI_UNIT(.MILLI.,.METRE.)
) ;
#4307=(
NAMED_UNIT(*)
PLANE_ANGLE_UNIT()
SI_UNIT($,.RADIAN.)
) ;
#4308=(
NAMED_UNIT(*)
SI_UNIT($,.STERADIAN.)
SOLID_ANGLE_UNIT()
) ;
#4310=SHAPE_DEFINITION_REPRESENTATION(#4315,#4331) ;
#4315=PRODUCT_DEFINITION_SHAPE('',$,#4337) ;
#4331=SHAPE_REPRESENTATION('',(#2214),#4300) ;
#4335=PRODUCT_DEFINITION_CONTEXT('part definition',#4352,'design') ;
#4337=PRODUCT_DEFINITION('Conjunction','Conjunction',#4342,#4335) ;
#4342=PRODUCT_DEFINITION_FORMATION('',$,#4355) ;
#4352=APPLICATION_CONTEXT(
'Core Data for Automotive Mechanical Design Process') ;
#4353=PRODUCT_CONTEXT('part definition',#4352,'mechanical') ;
#4355=PRODUCT('Conjunction','Conjunction',$,(#4353)) ;
#4360=PRESENTATION_STYLE_ASSIGNMENT((#4364)) ;
#4364=SURFACE_STYLE_USAGE(.BOTH.,#4368) ;
#4368=SURFACE_SIDE_STYLE('',(#4372)) ;
#4372=SURFACE_STYLE_FILL_AREA(#4376) ;
#4376=FILL_AREA_STYLE('Opaque(243,203,124)',(#4380)) ;
#4380=FILL_AREA_STYLE_COLOUR('Opaque(243,203,124)',#4384) ;
#4384=COLOUR_RGB('Opaque(243,203,124)', 0.09019608, 0.27058824, 0.51372549) ;
ENDSEC;
END-ISO-10303-21;
